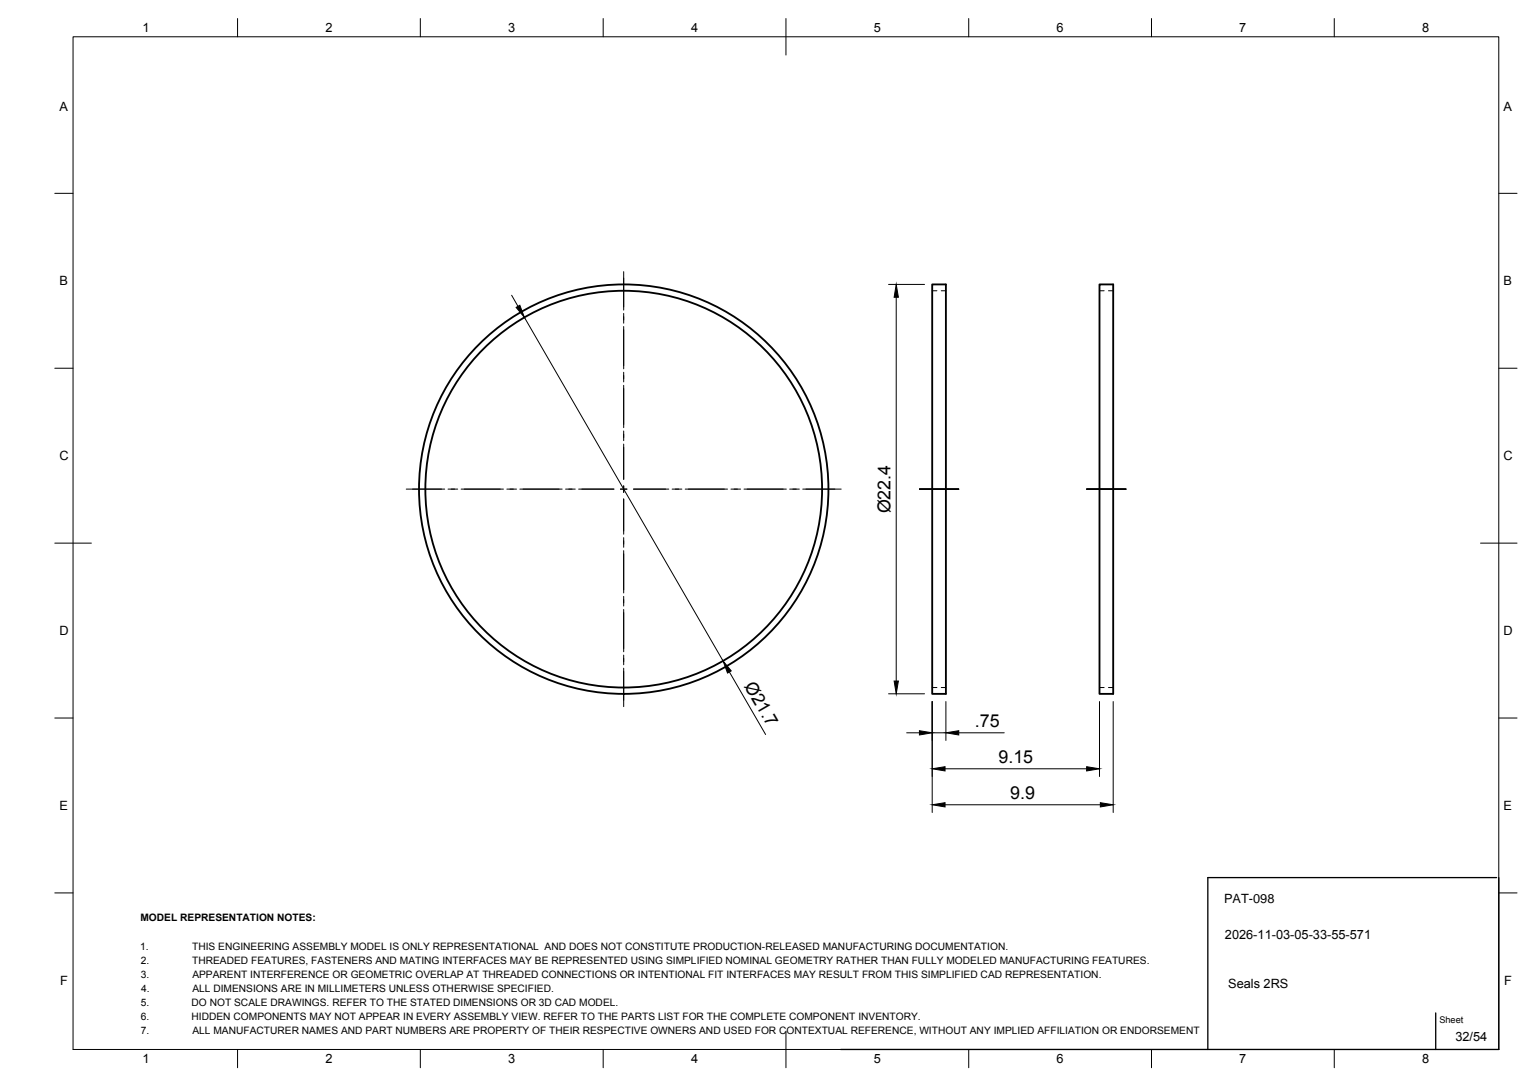
ISO-10303-21;
HEADER;
/* Generated by software containing ST-Developer
 * from STEP Tools, Inc. (www.steptools.com) 
 */

FILE_DESCRIPTION(
/* description */ ('Spring compression tester'),
/* implementation_level */ '2;1');

FILE_NAME(
/* name */ 'Seals 2RS.step',
/* time_stamp */ '2026-10-28T03:24:11-07:00',
/* author */ (''),
/* organization */ (''),
/* preprocessor_version */ 'ST-DEVELOPER v20.2',
/* originating_system */ 'Autodesk Translation Framework v15.17.0.0',
/* authorisation */ '');

FILE_SCHEMA (('AUTOMOTIVE_DESIGN { 1 0 10303 214 3 1 1 }'));
ENDSEC;

DATA;
#10=MECHANICAL_DESIGN_GEOMETRIC_PRESENTATION_REPRESENTATION('',(#1137,#1138),#43521);
#1011=SHAPE_REPRESENTATION_RELATIONSHIP('SRR','None',#43824,#1071);
#1071=ADVANCED_BREP_SHAPE_REPRESENTATION('',(#1211,#1212),#43484);
#1137=STYLED_ITEM('',(#44202),#1211);
#1138=STYLED_ITEM('',(#44202),#1212);
#1211=MANIFOLD_SOLID_BREP('Body1',#18575);
#1212=MANIFOLD_SOLID_BREP('Body2',#18576);
#1455=FACE_BOUND('',#3892,.T.);
#1456=FACE_BOUND('',#3895,.T.);
#1457=FACE_BOUND('',#3898,.T.);
#1458=FACE_BOUND('',#3901,.T.);
#1900=PLANE('',#20099);
#1901=PLANE('',#20104);
#1902=PLANE('',#20107);
#1903=PLANE('',#20112);
#2636=FACE_OUTER_BOUND('',#3891,.T.);
#2637=FACE_OUTER_BOUND('',#3893,.T.);
#2638=FACE_OUTER_BOUND('',#3894,.T.);
#2639=FACE_OUTER_BOUND('',#3896,.T.);
#2640=FACE_OUTER_BOUND('',#3897,.T.);
#2641=FACE_OUTER_BOUND('',#3899,.T.);
#2642=FACE_OUTER_BOUND('',#3900,.T.);
#2643=FACE_OUTER_BOUND('',#3902,.T.);
#3891=EDGE_LOOP('',(#14295));
#3892=EDGE_LOOP('',(#14296));
#3893=EDGE_LOOP('',(#14297,#14298,#14299,#14300));
#3894=EDGE_LOOP('',(#14301));
#3895=EDGE_LOOP('',(#14302));
#3896=EDGE_LOOP('',(#14303,#14304,#14305,#14306));
#3897=EDGE_LOOP('',(#14307));
#3898=EDGE_LOOP('',(#14308));
#3899=EDGE_LOOP('',(#14309,#14310,#14311,#14312));
#3900=EDGE_LOOP('',(#14313));
#3901=EDGE_LOOP('',(#14314));
#3902=EDGE_LOOP('',(#14315,#14316,#14317,#14318));
#5313=LINE('',#28989,#6745);
#5314=LINE('',#28994,#6746);
#5315=LINE('',#29003,#6747);
#5316=LINE('',#29008,#6748);
#6745=VECTOR('',#23543,1.119765);
#6746=VECTOR('',#23550,1.085235);
#6747=VECTOR('',#23561,1.119765);
#6748=VECTOR('',#23568,1.085235);
#7788=CIRCLE('',#20100,1.119765);
#7789=CIRCLE('',#20101,1.085235);
#7790=CIRCLE('',#20103,1.119765);
#7791=CIRCLE('',#20105,1.085235);
#7792=CIRCLE('',#20108,1.119765);
#7793=CIRCLE('',#20109,1.085235);
#7794=CIRCLE('',#20111,1.119765);
#7795=CIRCLE('',#20113,1.085235);
#8835=VERTEX_POINT('',#28982);
#8836=VERTEX_POINT('',#28984);
#8837=VERTEX_POINT('',#28987);
#8838=VERTEX_POINT('',#28991);
#8839=VERTEX_POINT('',#28996);
#8840=VERTEX_POINT('',#28998);
#8841=VERTEX_POINT('',#29001);
#8842=VERTEX_POINT('',#29005);
#10812=EDGE_CURVE('',#8835,#8835,#7788,.T.);
#10813=EDGE_CURVE('',#8836,#8836,#7789,.T.);
#10814=EDGE_CURVE('',#8837,#8837,#7790,.T.);
#10815=EDGE_CURVE('',#8837,#8835,#5313,.T.);
#10816=EDGE_CURVE('',#8838,#8838,#7791,.T.);
#10817=EDGE_CURVE('',#8838,#8836,#5314,.T.);
#10818=EDGE_CURVE('',#8839,#8839,#7792,.T.);
#10819=EDGE_CURVE('',#8840,#8840,#7793,.T.);
#10820=EDGE_CURVE('',#8841,#8841,#7794,.T.);
#10821=EDGE_CURVE('',#8841,#8839,#5315,.T.);
#10822=EDGE_CURVE('',#8842,#8842,#7795,.T.);
#10823=EDGE_CURVE('',#8842,#8840,#5316,.T.);
#14295=ORIENTED_EDGE('',*,*,#10812,.F.);
#14296=ORIENTED_EDGE('',*,*,#10813,.T.);
#14297=ORIENTED_EDGE('',*,*,#10814,.F.);
#14298=ORIENTED_EDGE('',*,*,#10815,.T.);
#14299=ORIENTED_EDGE('',*,*,#10812,.T.);
#14300=ORIENTED_EDGE('',*,*,#10815,.F.);
#14301=ORIENTED_EDGE('',*,*,#10814,.T.);
#14302=ORIENTED_EDGE('',*,*,#10816,.F.);
#14303=ORIENTED_EDGE('',*,*,#10816,.T.);
#14304=ORIENTED_EDGE('',*,*,#10817,.T.);
#14305=ORIENTED_EDGE('',*,*,#10813,.F.);
#14306=ORIENTED_EDGE('',*,*,#10817,.F.);
#14307=ORIENTED_EDGE('',*,*,#10818,.F.);
#14308=ORIENTED_EDGE('',*,*,#10819,.T.);
#14309=ORIENTED_EDGE('',*,*,#10820,.F.);
#14310=ORIENTED_EDGE('',*,*,#10821,.T.);
#14311=ORIENTED_EDGE('',*,*,#10818,.T.);
#14312=ORIENTED_EDGE('',*,*,#10821,.F.);
#14313=ORIENTED_EDGE('',*,*,#10820,.T.);
#14314=ORIENTED_EDGE('',*,*,#10822,.F.);
#14315=ORIENTED_EDGE('',*,*,#10822,.T.);
#14316=ORIENTED_EDGE('',*,*,#10823,.T.);
#14317=ORIENTED_EDGE('',*,*,#10819,.F.);
#14318=ORIENTED_EDGE('',*,*,#10823,.F.);
#17235=CYLINDRICAL_SURFACE('',#20102,1.119765);
#17236=CYLINDRICAL_SURFACE('',#20106,1.085235);
#17237=CYLINDRICAL_SURFACE('',#20110,1.119765);
#17238=CYLINDRICAL_SURFACE('',#20114,1.085235);
#17960=ADVANCED_FACE('',(#2636,#1455),#1900,.T.);
#17961=ADVANCED_FACE('',(#2637),#17235,.T.);
#17962=ADVANCED_FACE('',(#2638,#1456),#1901,.T.);
#17963=ADVANCED_FACE('',(#2639),#17236,.F.);
#17964=ADVANCED_FACE('',(#2640,#1457),#1902,.T.);
#17965=ADVANCED_FACE('',(#2641),#17237,.T.);
#17966=ADVANCED_FACE('',(#2642,#1458),#1903,.T.);
#17967=ADVANCED_FACE('',(#2643),#17238,.F.);
#18575=CLOSED_SHELL('',(#17960,#17961,#17962,#17963));
#18576=CLOSED_SHELL('',(#17964,#17965,#17966,#17967));
#20098=AXIS2_PLACEMENT_3D('',#28980,#23531,#23532);
#20099=AXIS2_PLACEMENT_3D('',#28981,#23533,#23534);
#20100=AXIS2_PLACEMENT_3D('',#28983,#23535,#23536);
#20101=AXIS2_PLACEMENT_3D('',#28985,#23537,#23538);
#20102=AXIS2_PLACEMENT_3D('',#28986,#23539,#23540);
#20103=AXIS2_PLACEMENT_3D('',#28988,#23541,#23542);
#20104=AXIS2_PLACEMENT_3D('',#28990,#23544,#23545);
#20105=AXIS2_PLACEMENT_3D('',#28992,#23546,#23547);
#20106=AXIS2_PLACEMENT_3D('',#28993,#23548,#23549);
#20107=AXIS2_PLACEMENT_3D('',#28995,#23551,#23552);
#20108=AXIS2_PLACEMENT_3D('',#28997,#23553,#23554);
#20109=AXIS2_PLACEMENT_3D('',#28999,#23555,#23556);
#20110=AXIS2_PLACEMENT_3D('',#29000,#23557,#23558);
#20111=AXIS2_PLACEMENT_3D('',#29002,#23559,#23560);
#20112=AXIS2_PLACEMENT_3D('',#29004,#23562,#23563);
#20113=AXIS2_PLACEMENT_3D('',#29006,#23564,#23565);
#20114=AXIS2_PLACEMENT_3D('',#29007,#23566,#23567);
#23531=DIRECTION('axis',(0.,0.,1.));
#23532=DIRECTION('refdir',(1.,0.,0.));
#23533=DIRECTION('center_axis',(0.,1.,0.));
#23534=DIRECTION('ref_axis',(0.,0.,1.));
#23535=DIRECTION('center_axis',(0.,-1.,0.));
#23536=DIRECTION('ref_axis',(1.,0.,0.));
#23537=DIRECTION('center_axis',(0.,-1.,0.));
#23538=DIRECTION('ref_axis',(1.,0.,0.));
#23539=DIRECTION('center_axis',(0.,-1.,0.));
#23540=DIRECTION('ref_axis',(1.,0.,0.));
#23541=DIRECTION('center_axis',(0.,-1.,0.));
#23542=DIRECTION('ref_axis',(1.,0.,0.));
#23543=DIRECTION('',(0.,1.,0.));
#23544=DIRECTION('center_axis',(0.,-1.,0.));
#23545=DIRECTION('ref_axis',(0.,0.,-1.));
#23546=DIRECTION('center_axis',(0.,-1.,0.));
#23547=DIRECTION('ref_axis',(1.,0.,0.));
#23548=DIRECTION('center_axis',(0.,-1.,0.));
#23549=DIRECTION('ref_axis',(1.,0.,0.));
#23550=DIRECTION('',(0.,1.,0.));
#23551=DIRECTION('center_axis',(0.,1.,0.));
#23552=DIRECTION('ref_axis',(0.,0.,1.));
#23553=DIRECTION('center_axis',(0.,-1.,0.));
#23554=DIRECTION('ref_axis',(1.,0.,0.));
#23555=DIRECTION('center_axis',(0.,-1.,0.));
#23556=DIRECTION('ref_axis',(1.,0.,0.));
#23557=DIRECTION('center_axis',(0.,-1.,0.));
#23558=DIRECTION('ref_axis',(1.,0.,0.));
#23559=DIRECTION('center_axis',(0.,-1.,0.));
#23560=DIRECTION('ref_axis',(1.,0.,0.));
#23561=DIRECTION('',(0.,1.,0.));
#23562=DIRECTION('center_axis',(0.,-1.,0.));
#23563=DIRECTION('ref_axis',(0.,0.,-1.));
#23564=DIRECTION('center_axis',(0.,-1.,0.));
#23565=DIRECTION('ref_axis',(1.,0.,0.));
#23566=DIRECTION('center_axis',(0.,-1.,0.));
#23567=DIRECTION('ref_axis',(1.,0.,0.));
#23568=DIRECTION('',(0.,1.,0.));
#28980=CARTESIAN_POINT('',(0.,0.,0.));
#28981=CARTESIAN_POINT('Origin',(1.119765,0.495,0.));
#28982=CARTESIAN_POINT('',(-1.119765,0.495,-1.37131662304724E-16));
#28983=CARTESIAN_POINT('Origin',(0.,0.495,0.));
#28984=CARTESIAN_POINT('',(-1.085235,0.495,-1.32902956907268E-16));
#28985=CARTESIAN_POINT('Origin',(0.,0.495,0.));
#28986=CARTESIAN_POINT('Origin',(0.,0.4575,0.));
#28987=CARTESIAN_POINT('',(-1.119765,0.42,-1.37131662304724E-16));
#28988=CARTESIAN_POINT('Origin',(0.,0.42,0.));
#28989=CARTESIAN_POINT('',(-1.119765,0.4575,-1.37131662304724E-16));
#28990=CARTESIAN_POINT('Origin',(1.085235,0.42,0.));
#28991=CARTESIAN_POINT('',(-1.085235,0.42,-1.32902956907268E-16));
#28992=CARTESIAN_POINT('Origin',(0.,0.42,0.));
#28993=CARTESIAN_POINT('Origin',(0.,0.4575,0.));
#28994=CARTESIAN_POINT('',(-1.085235,0.4575,-1.32902956907268E-16));
#28995=CARTESIAN_POINT('Origin',(1.119765,-0.42,0.));
#28996=CARTESIAN_POINT('',(-1.119765,-0.42,-1.37131662304724E-16));
#28997=CARTESIAN_POINT('Origin',(0.,-0.42,0.));
#28998=CARTESIAN_POINT('',(-1.085235,-0.42,-1.32902956907268E-16));
#28999=CARTESIAN_POINT('Origin',(0.,-0.42,0.));
#29000=CARTESIAN_POINT('Origin',(0.,-0.4575,0.));
#29001=CARTESIAN_POINT('',(-1.119765,-0.495,-1.37131662304724E-16));
#29002=CARTESIAN_POINT('Origin',(0.,-0.495,0.));
#29003=CARTESIAN_POINT('',(-1.119765,-0.4575,-1.37131662304724E-16));
#29004=CARTESIAN_POINT('Origin',(1.085235,-0.495,0.));
#29005=CARTESIAN_POINT('',(-1.085235,-0.495,-1.32902956907268E-16));
#29006=CARTESIAN_POINT('Origin',(0.,-0.495,0.));
#29007=CARTESIAN_POINT('Origin',(0.,-0.4575,0.));
#29008=CARTESIAN_POINT('',(-1.085235,-0.4575,-1.32902956907268E-16));
#43416=UNCERTAINTY_MEASURE_WITH_UNIT(LENGTH_MEASURE(0.001),#43522,
'DISTANCE_ACCURACY_VALUE',
'Maximum model space distance between geometric entities at asserted c
onnectivities');
#43453=UNCERTAINTY_MEASURE_WITH_UNIT(LENGTH_MEASURE(0.001),#43522,
'DISTANCE_ACCURACY_VALUE',
'Maximum model space distance between geometric entities at asserted c
onnectivities');
#43484=(
GEOMETRIC_REPRESENTATION_CONTEXT(3)
GLOBAL_UNCERTAINTY_ASSIGNED_CONTEXT((#43416))
GLOBAL_UNIT_ASSIGNED_CONTEXT((#43522,#43524,#43525))
REPRESENTATION_CONTEXT('','3D')
);
#43521=(
GEOMETRIC_REPRESENTATION_CONTEXT(3)
GLOBAL_UNCERTAINTY_ASSIGNED_CONTEXT((#43453))
GLOBAL_UNIT_ASSIGNED_CONTEXT((#43522,#43524,#43525))
REPRESENTATION_CONTEXT('','3D')
);
#43522=(
LENGTH_UNIT()
NAMED_UNIT(*)
SI_UNIT(.CENTI.,.METRE.)
);
#43524=(
NAMED_UNIT(*)
PLANE_ANGLE_UNIT()
SI_UNIT($,.RADIAN.)
);
#43525=(
NAMED_UNIT(*)
SI_UNIT($,.STERADIAN.)
SOLID_ANGLE_UNIT()
);
#43556=SHAPE_DEFINITION_REPRESENTATION(#43623,#43824);
#43623=PRODUCT_DEFINITION_SHAPE('',$,#43892);
#43824=SHAPE_REPRESENTATION('',(#20098),#43484);
#43861=PRODUCT_DEFINITION_CONTEXT('part definition',#44064,'design');
#43892=PRODUCT_DEFINITION('Seals 2RS','Seals 2RS',#43959,#43861);
#43959=PRODUCT_DEFINITION_FORMATION('',$,#44096);
#44064=APPLICATION_CONTEXT(
'Core Data for Automotive Mechanical Design Process');
#44065=PRODUCT_CONTEXT('part definition',#44064,'mechanical');
#44096=PRODUCT('Seals 2RS','Seals 2RS','Seals 2RS',(#44065));
#44196=COLOUR_RGB('Grey',0.48,0.52,0.57);
#44197=FILL_AREA_STYLE_COLOUR('',#44196);
#44198=FILL_AREA_STYLE('',(#44197));
#44199=SURFACE_STYLE_FILL_AREA(#44198);
#44200=SURFACE_SIDE_STYLE('',(#44199));
#44201=SURFACE_STYLE_USAGE(.BOTH.,#44200);
#44202=PRESENTATION_STYLE_ASSIGNMENT((#44201));
ENDSEC;
END-ISO-10303-21;
